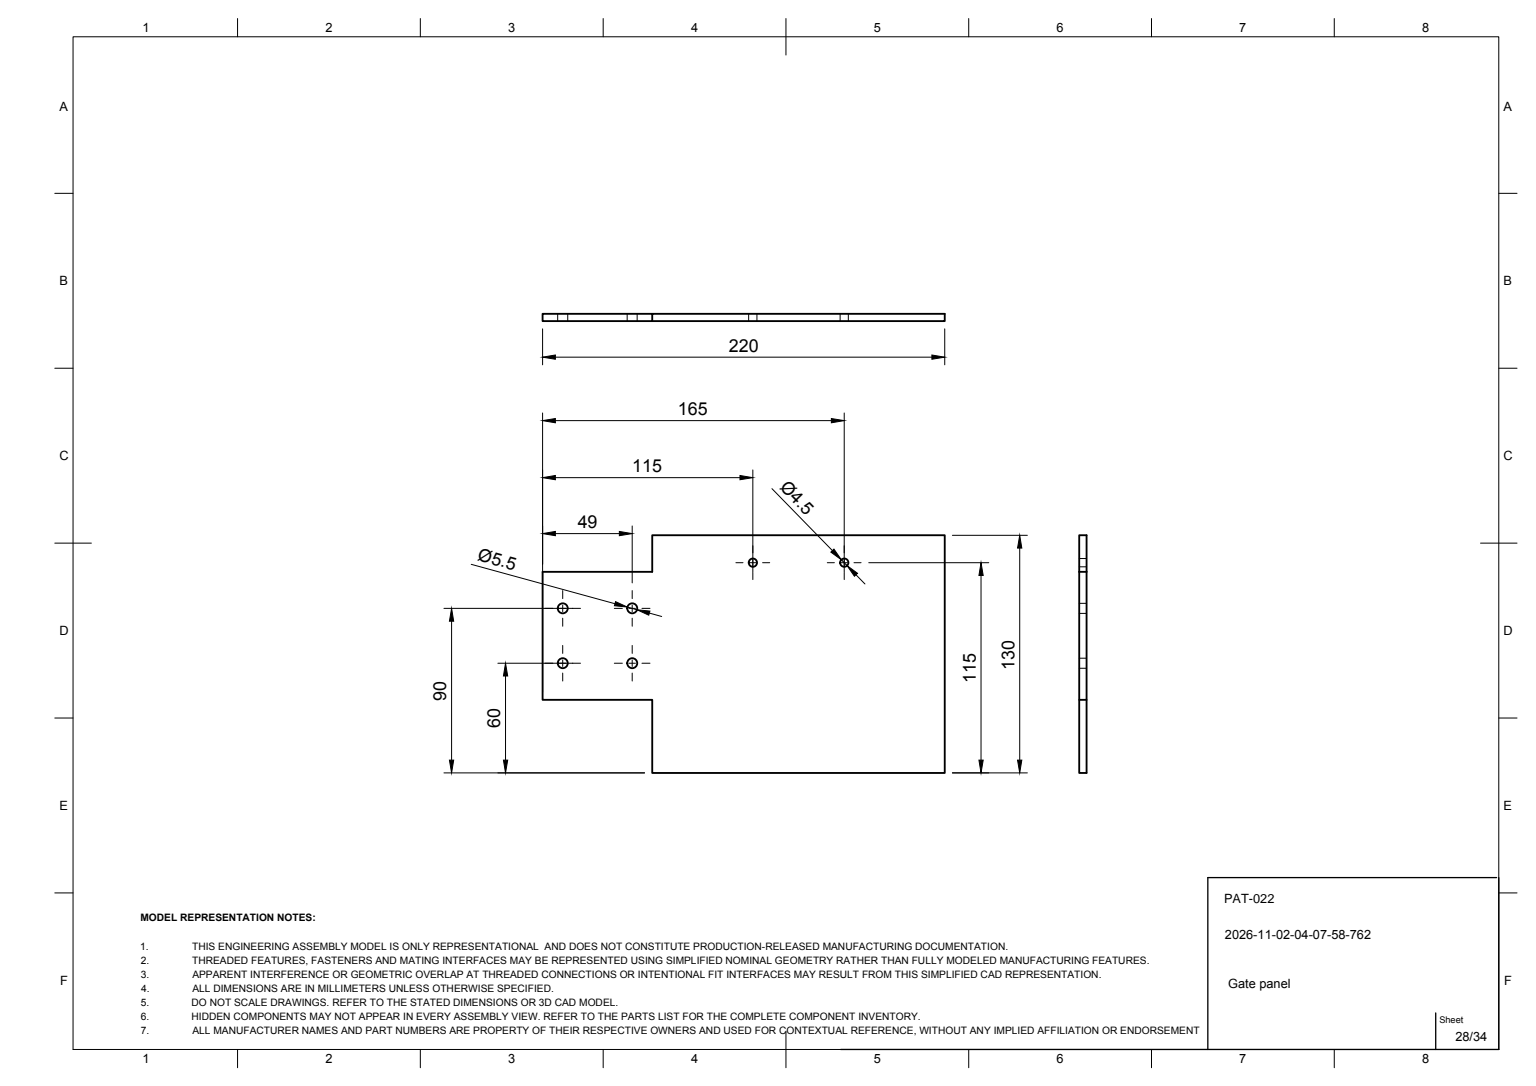
ISO-10303-21;
HEADER;
/* Generated by software containing ST-Developer
 * from STEP Tools, Inc. (www.steptools.com) 
 */

FILE_DESCRIPTION(
/* description */ ('Chute with adjustable gate'),
/* implementation_level */ '2;1');

FILE_NAME(
/* name */ 'Gate panel.step',
/* time_stamp */ '2026-10-27T10:52:28-07:00',
/* author */ (''),
/* organization */ (''),
/* preprocessor_version */ 'ST-DEVELOPER v20.2',
/* originating_system */ 'Autodesk Translation Framework v15.17.0.0',
/* authorisation */ '');

FILE_SCHEMA (('AUTOMOTIVE_DESIGN { 1 0 10303 214 3 1 1 }'));
ENDSEC;

DATA;
#10=MECHANICAL_DESIGN_GEOMETRIC_PRESENTATION_REPRESENTATION('',(#439),#13094);
#375=SHAPE_REPRESENTATION_RELATIONSHIP('SRR','None',#13277,#407);
#407=ADVANCED_BREP_SHAPE_REPRESENTATION('',(#469),#13086);
#439=STYLED_ITEM('',(#13488),#469);
#469=MANIFOLD_SOLID_BREP('Body1',#7624);
#570=FACE_BOUND('',#1746,.T.);
#571=FACE_BOUND('',#1747,.T.);
#572=FACE_BOUND('',#1748,.T.);
#573=FACE_BOUND('',#1749,.T.);
#574=FACE_BOUND('',#1750,.T.);
#575=FACE_BOUND('',#1751,.T.);
#576=FACE_BOUND('',#1758,.T.);
#577=FACE_BOUND('',#1759,.T.);
#578=FACE_BOUND('',#1760,.T.);
#579=FACE_BOUND('',#1761,.T.);
#580=FACE_BOUND('',#1762,.T.);
#581=FACE_BOUND('',#1763,.T.);
#836=PLANE('',#8470);
#837=PLANE('',#8471);
#838=PLANE('',#8472);
#839=PLANE('',#8473);
#840=PLANE('',#8474);
#841=PLANE('',#8475);
#842=PLANE('',#8476);
#843=PLANE('',#8477);
#844=PLANE('',#8478);
#845=PLANE('',#8479);
#1225=FACE_OUTER_BOUND('',#1736,.T.);
#1226=FACE_OUTER_BOUND('',#1737,.T.);
#1227=FACE_OUTER_BOUND('',#1738,.T.);
#1228=FACE_OUTER_BOUND('',#1739,.T.);
#1229=FACE_OUTER_BOUND('',#1740,.T.);
#1230=FACE_OUTER_BOUND('',#1741,.T.);
#1231=FACE_OUTER_BOUND('',#1742,.T.);
#1232=FACE_OUTER_BOUND('',#1743,.T.);
#1233=FACE_OUTER_BOUND('',#1744,.T.);
#1234=FACE_OUTER_BOUND('',#1745,.T.);
#1235=FACE_OUTER_BOUND('',#1752,.T.);
#1236=FACE_OUTER_BOUND('',#1753,.T.);
#1237=FACE_OUTER_BOUND('',#1754,.T.);
#1238=FACE_OUTER_BOUND('',#1755,.T.);
#1239=FACE_OUTER_BOUND('',#1756,.T.);
#1240=FACE_OUTER_BOUND('',#1757,.T.);
#1736=EDGE_LOOP('',(#6616,#6617,#6618,#6619));
#1737=EDGE_LOOP('',(#6620,#6621,#6622,#6623));
#1738=EDGE_LOOP('',(#6624,#6625,#6626,#6627));
#1739=EDGE_LOOP('',(#6628,#6629,#6630,#6631));
#1740=EDGE_LOOP('',(#6632,#6633,#6634,#6635));
#1741=EDGE_LOOP('',(#6636,#6637,#6638,#6639));
#1742=EDGE_LOOP('',(#6640,#6641,#6642,#6643));
#1743=EDGE_LOOP('',(#6644,#6645,#6646,#6647));
#1744=EDGE_LOOP('',(#6648,#6649,#6650,#6651));
#1745=EDGE_LOOP('',(#6652,#6653,#6654,#6655,#6656,#6657,#6658,#6659));
#1746=EDGE_LOOP('',(#6660));
#1747=EDGE_LOOP('',(#6661));
#1748=EDGE_LOOP('',(#6662));
#1749=EDGE_LOOP('',(#6663));
#1750=EDGE_LOOP('',(#6664));
#1751=EDGE_LOOP('',(#6665));
#1752=EDGE_LOOP('',(#6666,#6667,#6668,#6669));
#1753=EDGE_LOOP('',(#6670,#6671,#6672,#6673));
#1754=EDGE_LOOP('',(#6674,#6675,#6676,#6677));
#1755=EDGE_LOOP('',(#6678,#6679,#6680,#6681));
#1756=EDGE_LOOP('',(#6682,#6683,#6684,#6685));
#1757=EDGE_LOOP('',(#6686,#6687,#6688,#6689,#6690,#6691,#6692,#6693));
#1758=EDGE_LOOP('',(#6694));
#1759=EDGE_LOOP('',(#6695));
#1760=EDGE_LOOP('',(#6696));
#1761=EDGE_LOOP('',(#6697));
#1762=EDGE_LOOP('',(#6698));
#1763=EDGE_LOOP('',(#6699));
#2449=LINE('',#12432,#3226);
#2450=LINE('',#12438,#3227);
#2451=LINE('',#12444,#3228);
#2452=LINE('',#12450,#3229);
#2453=LINE('',#12456,#3230);
#2454=LINE('',#12462,#3231);
#2455=LINE('',#12467,#3232);
#2456=LINE('',#12469,#3233);
#2457=LINE('',#12471,#3234);
#2458=LINE('',#12472,#3235);
#2459=LINE('',#12476,#3236);
#2460=LINE('',#12478,#3237);
#2461=LINE('',#12480,#3238);
#2462=LINE('',#12481,#3239);
#2463=LINE('',#12483,#3240);
#2464=LINE('',#12484,#3241);
#2465=LINE('',#12487,#3242);
#2466=LINE('',#12489,#3243);
#2467=LINE('',#12491,#3244);
#2468=LINE('',#12493,#3245);
#2469=LINE('',#12494,#3246);
#2470=LINE('',#12497,#3247);
#2471=LINE('',#12498,#3248);
#2472=LINE('',#12501,#3249);
#2473=LINE('',#12503,#3250);
#2474=LINE('',#12504,#3251);
#2475=LINE('',#12506,#3252);
#2476=LINE('',#12509,#3253);
#2477=LINE('',#12510,#3254);
#2478=LINE('',#12512,#3255);
#3226=VECTOR('',#10223,0.225);
#3227=VECTOR('',#10230,0.225);
#3228=VECTOR('',#10237,0.275);
#3229=VECTOR('',#10244,0.275);
#3230=VECTOR('',#10251,0.275);
#3231=VECTOR('',#10258,0.275);
#3232=VECTOR('',#10263,1.);
#3233=VECTOR('',#10264,1.);
#3234=VECTOR('',#10265,1.);
#3235=VECTOR('',#10266,1.);
#3236=VECTOR('',#10269,1.);
#3237=VECTOR('',#10270,1.);
#3238=VECTOR('',#10271,1.);
#3239=VECTOR('',#10272,1.);
#3240=VECTOR('',#10275,1.);
#3241=VECTOR('',#10276,1.);
#3242=VECTOR('',#10279,1.);
#3243=VECTOR('',#10280,1.);
#3244=VECTOR('',#10281,1.);
#3245=VECTOR('',#10282,1.);
#3246=VECTOR('',#10283,1.);
#3247=VECTOR('',#10286,1.);
#3248=VECTOR('',#10287,1.);
#3249=VECTOR('',#10290,1.);
#3250=VECTOR('',#10291,1.);
#3251=VECTOR('',#10292,1.);
#3252=VECTOR('',#10295,1.);
#3253=VECTOR('',#10298,1.);
#3254=VECTOR('',#10299,1.);
#3255=VECTOR('',#10302,1.);
#3538=CIRCLE('',#8453,0.225);
#3539=CIRCLE('',#8454,0.225);
#3540=CIRCLE('',#8456,0.225);
#3541=CIRCLE('',#8457,0.225);
#3542=CIRCLE('',#8459,0.275);
#3543=CIRCLE('',#8460,0.275);
#3544=CIRCLE('',#8462,0.275);
#3545=CIRCLE('',#8463,0.275);
#3546=CIRCLE('',#8465,0.275);
#3547=CIRCLE('',#8466,0.275);
#3548=CIRCLE('',#8468,0.275);
#3549=CIRCLE('',#8469,0.275);
#4067=VERTEX_POINT('',#12429);
#4068=VERTEX_POINT('',#12431);
#4069=VERTEX_POINT('',#12435);
#4070=VERTEX_POINT('',#12437);
#4071=VERTEX_POINT('',#12441);
#4072=VERTEX_POINT('',#12443);
#4073=VERTEX_POINT('',#12447);
#4074=VERTEX_POINT('',#12449);
#4075=VERTEX_POINT('',#12453);
#4076=VERTEX_POINT('',#12455);
#4077=VERTEX_POINT('',#12459);
#4078=VERTEX_POINT('',#12461);
#4079=VERTEX_POINT('',#12465);
#4080=VERTEX_POINT('',#12466);
#4081=VERTEX_POINT('',#12468);
#4082=VERTEX_POINT('',#12470);
#4083=VERTEX_POINT('',#12474);
#4084=VERTEX_POINT('',#12475);
#4085=VERTEX_POINT('',#12477);
#4086=VERTEX_POINT('',#12479);
#4087=VERTEX_POINT('',#12486);
#4088=VERTEX_POINT('',#12488);
#4089=VERTEX_POINT('',#12490);
#4090=VERTEX_POINT('',#12492);
#4091=VERTEX_POINT('',#12496);
#4092=VERTEX_POINT('',#12500);
#4093=VERTEX_POINT('',#12502);
#4094=VERTEX_POINT('',#12508);
#4941=EDGE_CURVE('',#4067,#4067,#3538,.T.);
#4942=EDGE_CURVE('',#4067,#4068,#2449,.T.);
#4943=EDGE_CURVE('',#4068,#4068,#3539,.T.);
#4944=EDGE_CURVE('',#4069,#4069,#3540,.T.);
#4945=EDGE_CURVE('',#4069,#4070,#2450,.T.);
#4946=EDGE_CURVE('',#4070,#4070,#3541,.T.);
#4947=EDGE_CURVE('',#4071,#4071,#3542,.T.);
#4948=EDGE_CURVE('',#4071,#4072,#2451,.T.);
#4949=EDGE_CURVE('',#4072,#4072,#3543,.T.);
#4950=EDGE_CURVE('',#4073,#4073,#3544,.T.);
#4951=EDGE_CURVE('',#4073,#4074,#2452,.T.);
#4952=EDGE_CURVE('',#4074,#4074,#3545,.T.);
#4953=EDGE_CURVE('',#4075,#4075,#3546,.T.);
#4954=EDGE_CURVE('',#4075,#4076,#2453,.T.);
#4955=EDGE_CURVE('',#4076,#4076,#3547,.T.);
#4956=EDGE_CURVE('',#4077,#4077,#3548,.T.);
#4957=EDGE_CURVE('',#4077,#4078,#2454,.T.);
#4958=EDGE_CURVE('',#4078,#4078,#3549,.T.);
#4959=EDGE_CURVE('',#4079,#4080,#2455,.T.);
#4960=EDGE_CURVE('',#4081,#4079,#2456,.T.);
#4961=EDGE_CURVE('',#4082,#4081,#2457,.T.);
#4962=EDGE_CURVE('',#4082,#4080,#2458,.T.);
#4963=EDGE_CURVE('',#4083,#4084,#2459,.T.);
#4964=EDGE_CURVE('',#4083,#4085,#2460,.T.);
#4965=EDGE_CURVE('',#4085,#4086,#2461,.T.);
#4966=EDGE_CURVE('',#4084,#4086,#2462,.T.);
#4967=EDGE_CURVE('',#4085,#4082,#2463,.T.);
#4968=EDGE_CURVE('',#4086,#4081,#2464,.T.);
#4969=EDGE_CURVE('',#4087,#4083,#2465,.T.);
#4970=EDGE_CURVE('',#4088,#4087,#2466,.T.);
#4971=EDGE_CURVE('',#4089,#4088,#2467,.T.);
#4972=EDGE_CURVE('',#4090,#4089,#2468,.T.);
#4973=EDGE_CURVE('',#4080,#4090,#2469,.T.);
#4974=EDGE_CURVE('',#4091,#4084,#2470,.T.);
#4975=EDGE_CURVE('',#4087,#4091,#2471,.T.);
#4976=EDGE_CURVE('',#4089,#4092,#2472,.T.);
#4977=EDGE_CURVE('',#4093,#4092,#2473,.T.);
#4978=EDGE_CURVE('',#4090,#4093,#2474,.T.);
#4979=EDGE_CURVE('',#4079,#4093,#2475,.T.);
#4980=EDGE_CURVE('',#4094,#4091,#2476,.T.);
#4981=EDGE_CURVE('',#4088,#4094,#2477,.T.);
#4982=EDGE_CURVE('',#4092,#4094,#2478,.T.);
#6616=ORIENTED_EDGE('',*,*,#4941,.F.);
#6617=ORIENTED_EDGE('',*,*,#4942,.T.);
#6618=ORIENTED_EDGE('',*,*,#4943,.F.);
#6619=ORIENTED_EDGE('',*,*,#4942,.F.);
#6620=ORIENTED_EDGE('',*,*,#4944,.F.);
#6621=ORIENTED_EDGE('',*,*,#4945,.T.);
#6622=ORIENTED_EDGE('',*,*,#4946,.F.);
#6623=ORIENTED_EDGE('',*,*,#4945,.F.);
#6624=ORIENTED_EDGE('',*,*,#4947,.F.);
#6625=ORIENTED_EDGE('',*,*,#4948,.T.);
#6626=ORIENTED_EDGE('',*,*,#4949,.F.);
#6627=ORIENTED_EDGE('',*,*,#4948,.F.);
#6628=ORIENTED_EDGE('',*,*,#4950,.F.);
#6629=ORIENTED_EDGE('',*,*,#4951,.T.);
#6630=ORIENTED_EDGE('',*,*,#4952,.F.);
#6631=ORIENTED_EDGE('',*,*,#4951,.F.);
#6632=ORIENTED_EDGE('',*,*,#4953,.F.);
#6633=ORIENTED_EDGE('',*,*,#4954,.T.);
#6634=ORIENTED_EDGE('',*,*,#4955,.F.);
#6635=ORIENTED_EDGE('',*,*,#4954,.F.);
#6636=ORIENTED_EDGE('',*,*,#4956,.F.);
#6637=ORIENTED_EDGE('',*,*,#4957,.T.);
#6638=ORIENTED_EDGE('',*,*,#4958,.F.);
#6639=ORIENTED_EDGE('',*,*,#4957,.F.);
#6640=ORIENTED_EDGE('',*,*,#4959,.F.);
#6641=ORIENTED_EDGE('',*,*,#4960,.F.);
#6642=ORIENTED_EDGE('',*,*,#4961,.F.);
#6643=ORIENTED_EDGE('',*,*,#4962,.T.);
#6644=ORIENTED_EDGE('',*,*,#4963,.F.);
#6645=ORIENTED_EDGE('',*,*,#4964,.T.);
#6646=ORIENTED_EDGE('',*,*,#4965,.T.);
#6647=ORIENTED_EDGE('',*,*,#4966,.F.);
#6648=ORIENTED_EDGE('',*,*,#4967,.T.);
#6649=ORIENTED_EDGE('',*,*,#4961,.T.);
#6650=ORIENTED_EDGE('',*,*,#4968,.F.);
#6651=ORIENTED_EDGE('',*,*,#4965,.F.);
#6652=ORIENTED_EDGE('',*,*,#4969,.F.);
#6653=ORIENTED_EDGE('',*,*,#4970,.F.);
#6654=ORIENTED_EDGE('',*,*,#4971,.F.);
#6655=ORIENTED_EDGE('',*,*,#4972,.F.);
#6656=ORIENTED_EDGE('',*,*,#4973,.F.);
#6657=ORIENTED_EDGE('',*,*,#4962,.F.);
#6658=ORIENTED_EDGE('',*,*,#4967,.F.);
#6659=ORIENTED_EDGE('',*,*,#4964,.F.);
#6660=ORIENTED_EDGE('',*,*,#4941,.T.);
#6661=ORIENTED_EDGE('',*,*,#4944,.T.);
#6662=ORIENTED_EDGE('',*,*,#4947,.T.);
#6663=ORIENTED_EDGE('',*,*,#4950,.T.);
#6664=ORIENTED_EDGE('',*,*,#4953,.T.);
#6665=ORIENTED_EDGE('',*,*,#4956,.T.);
#6666=ORIENTED_EDGE('',*,*,#4963,.T.);
#6667=ORIENTED_EDGE('',*,*,#4974,.F.);
#6668=ORIENTED_EDGE('',*,*,#4975,.F.);
#6669=ORIENTED_EDGE('',*,*,#4969,.T.);
#6670=ORIENTED_EDGE('',*,*,#4972,.T.);
#6671=ORIENTED_EDGE('',*,*,#4976,.T.);
#6672=ORIENTED_EDGE('',*,*,#4977,.F.);
#6673=ORIENTED_EDGE('',*,*,#4978,.F.);
#6674=ORIENTED_EDGE('',*,*,#4959,.T.);
#6675=ORIENTED_EDGE('',*,*,#4973,.T.);
#6676=ORIENTED_EDGE('',*,*,#4978,.T.);
#6677=ORIENTED_EDGE('',*,*,#4979,.F.);
#6678=ORIENTED_EDGE('',*,*,#4970,.T.);
#6679=ORIENTED_EDGE('',*,*,#4975,.T.);
#6680=ORIENTED_EDGE('',*,*,#4980,.F.);
#6681=ORIENTED_EDGE('',*,*,#4981,.F.);
#6682=ORIENTED_EDGE('',*,*,#4971,.T.);
#6683=ORIENTED_EDGE('',*,*,#4981,.T.);
#6684=ORIENTED_EDGE('',*,*,#4982,.F.);
#6685=ORIENTED_EDGE('',*,*,#4976,.F.);
#6686=ORIENTED_EDGE('',*,*,#4979,.T.);
#6687=ORIENTED_EDGE('',*,*,#4977,.T.);
#6688=ORIENTED_EDGE('',*,*,#4982,.T.);
#6689=ORIENTED_EDGE('',*,*,#4980,.T.);
#6690=ORIENTED_EDGE('',*,*,#4974,.T.);
#6691=ORIENTED_EDGE('',*,*,#4966,.T.);
#6692=ORIENTED_EDGE('',*,*,#4968,.T.);
#6693=ORIENTED_EDGE('',*,*,#4960,.T.);
#6694=ORIENTED_EDGE('',*,*,#4943,.T.);
#6695=ORIENTED_EDGE('',*,*,#4946,.T.);
#6696=ORIENTED_EDGE('',*,*,#4949,.T.);
#6697=ORIENTED_EDGE('',*,*,#4952,.T.);
#6698=ORIENTED_EDGE('',*,*,#4955,.T.);
#6699=ORIENTED_EDGE('',*,*,#4958,.T.);
#7163=CYLINDRICAL_SURFACE('',#8452,0.225);
#7164=CYLINDRICAL_SURFACE('',#8455,0.225);
#7165=CYLINDRICAL_SURFACE('',#8458,0.275);
#7166=CYLINDRICAL_SURFACE('',#8461,0.275);
#7167=CYLINDRICAL_SURFACE('',#8464,0.275);
#7168=CYLINDRICAL_SURFACE('',#8467,0.275);
#7493=ADVANCED_FACE('',(#1225),#7163,.F.);
#7494=ADVANCED_FACE('',(#1226),#7164,.F.);
#7495=ADVANCED_FACE('',(#1227),#7165,.F.);
#7496=ADVANCED_FACE('',(#1228),#7166,.F.);
#7497=ADVANCED_FACE('',(#1229),#7167,.F.);
#7498=ADVANCED_FACE('',(#1230),#7168,.F.);
#7499=ADVANCED_FACE('',(#1231),#836,.T.);
#7500=ADVANCED_FACE('',(#1232),#837,.T.);
#7501=ADVANCED_FACE('',(#1233),#838,.T.);
#7502=ADVANCED_FACE('',(#1234,#570,#571,#572,#573,#574,#575),#839,.F.);
#7503=ADVANCED_FACE('',(#1235),#840,.T.);
#7504=ADVANCED_FACE('',(#1236),#841,.T.);
#7505=ADVANCED_FACE('',(#1237),#842,.T.);
#7506=ADVANCED_FACE('',(#1238),#843,.T.);
#7507=ADVANCED_FACE('',(#1239),#844,.T.);
#7508=ADVANCED_FACE('',(#1240,#576,#577,#578,#579,#580,#581),#845,.T.);
#7624=CLOSED_SHELL('',(#7493,#7494,#7495,#7496,#7497,#7498,#7499,#7500,
#7501,#7502,#7503,#7504,#7505,#7506,#7507,#7508));
#8451=AXIS2_PLACEMENT_3D('',#12427,#10217,#10218);
#8452=AXIS2_PLACEMENT_3D('',#12428,#10219,#10220);
#8453=AXIS2_PLACEMENT_3D('',#12430,#10221,#10222);
#8454=AXIS2_PLACEMENT_3D('',#12433,#10224,#10225);
#8455=AXIS2_PLACEMENT_3D('',#12434,#10226,#10227);
#8456=AXIS2_PLACEMENT_3D('',#12436,#10228,#10229);
#8457=AXIS2_PLACEMENT_3D('',#12439,#10231,#10232);
#8458=AXIS2_PLACEMENT_3D('',#12440,#10233,#10234);
#8459=AXIS2_PLACEMENT_3D('',#12442,#10235,#10236);
#8460=AXIS2_PLACEMENT_3D('',#12445,#10238,#10239);
#8461=AXIS2_PLACEMENT_3D('',#12446,#10240,#10241);
#8462=AXIS2_PLACEMENT_3D('',#12448,#10242,#10243);
#8463=AXIS2_PLACEMENT_3D('',#12451,#10245,#10246);
#8464=AXIS2_PLACEMENT_3D('',#12452,#10247,#10248);
#8465=AXIS2_PLACEMENT_3D('',#12454,#10249,#10250);
#8466=AXIS2_PLACEMENT_3D('',#12457,#10252,#10253);
#8467=AXIS2_PLACEMENT_3D('',#12458,#10254,#10255);
#8468=AXIS2_PLACEMENT_3D('',#12460,#10256,#10257);
#8469=AXIS2_PLACEMENT_3D('',#12463,#10259,#10260);
#8470=AXIS2_PLACEMENT_3D('',#12464,#10261,#10262);
#8471=AXIS2_PLACEMENT_3D('',#12473,#10267,#10268);
#8472=AXIS2_PLACEMENT_3D('',#12482,#10273,#10274);
#8473=AXIS2_PLACEMENT_3D('',#12485,#10277,#10278);
#8474=AXIS2_PLACEMENT_3D('',#12495,#10284,#10285);
#8475=AXIS2_PLACEMENT_3D('',#12499,#10288,#10289);
#8476=AXIS2_PLACEMENT_3D('',#12505,#10293,#10294);
#8477=AXIS2_PLACEMENT_3D('',#12507,#10296,#10297);
#8478=AXIS2_PLACEMENT_3D('',#12511,#10300,#10301);
#8479=AXIS2_PLACEMENT_3D('',#12513,#10303,#10304);
#10217=DIRECTION('axis',(0.,0.,1.));
#10218=DIRECTION('refdir',(1.,0.,0.));
#10219=DIRECTION('center_axis',(1.,0.,0.));
#10220=DIRECTION('ref_axis',(0.,0.,-1.));
#10221=DIRECTION('center_axis',(1.,0.,0.));
#10222=DIRECTION('ref_axis',(0.,0.,-1.));
#10223=DIRECTION('',(1.,0.,0.));
#10224=DIRECTION('center_axis',(-1.,0.,0.));
#10225=DIRECTION('ref_axis',(0.,0.,-1.));
#10226=DIRECTION('center_axis',(1.,0.,0.));
#10227=DIRECTION('ref_axis',(0.,0.,-1.));
#10228=DIRECTION('center_axis',(1.,0.,0.));
#10229=DIRECTION('ref_axis',(0.,0.,-1.));
#10230=DIRECTION('',(1.,0.,0.));
#10231=DIRECTION('center_axis',(-1.,0.,0.));
#10232=DIRECTION('ref_axis',(0.,0.,-1.));
#10233=DIRECTION('center_axis',(1.,0.,0.));
#10234=DIRECTION('ref_axis',(0.,0.,-1.));
#10235=DIRECTION('center_axis',(1.,0.,0.));
#10236=DIRECTION('ref_axis',(0.,0.,-1.));
#10237=DIRECTION('',(1.,0.,0.));
#10238=DIRECTION('center_axis',(-1.,0.,0.));
#10239=DIRECTION('ref_axis',(0.,0.,-1.));
#10240=DIRECTION('center_axis',(1.,0.,0.));
#10241=DIRECTION('ref_axis',(0.,0.,-1.));
#10242=DIRECTION('center_axis',(1.,0.,0.));
#10243=DIRECTION('ref_axis',(0.,0.,-1.));
#10244=DIRECTION('',(1.,0.,0.));
#10245=DIRECTION('center_axis',(-1.,0.,0.));
#10246=DIRECTION('ref_axis',(0.,0.,-1.));
#10247=DIRECTION('center_axis',(1.,0.,0.));
#10248=DIRECTION('ref_axis',(0.,0.,-1.));
#10249=DIRECTION('center_axis',(1.,0.,0.));
#10250=DIRECTION('ref_axis',(0.,0.,-1.));
#10251=DIRECTION('',(1.,0.,0.));
#10252=DIRECTION('center_axis',(-1.,0.,0.));
#10253=DIRECTION('ref_axis',(0.,0.,-1.));
#10254=DIRECTION('center_axis',(1.,0.,0.));
#10255=DIRECTION('ref_axis',(0.,0.,-1.));
#10256=DIRECTION('center_axis',(1.,0.,0.));
#10257=DIRECTION('ref_axis',(0.,0.,-1.));
#10258=DIRECTION('',(1.,0.,0.));
#10259=DIRECTION('center_axis',(-1.,0.,0.));
#10260=DIRECTION('ref_axis',(0.,0.,-1.));
#10261=DIRECTION('center_axis',(0.,0.,1.));
#10262=DIRECTION('ref_axis',(0.,-1.,0.));
#10263=DIRECTION('',(-1.,0.,0.));
#10264=DIRECTION('',(0.,-1.,0.));
#10265=DIRECTION('',(1.,0.,0.));
#10266=DIRECTION('',(0.,-1.,0.));
#10267=DIRECTION('center_axis',(0.,0.,-1.));
#10268=DIRECTION('ref_axis',(0.,1.,0.));
#10269=DIRECTION('',(1.,0.,0.));
#10270=DIRECTION('',(0.,1.,0.));
#10271=DIRECTION('',(1.,0.,0.));
#10272=DIRECTION('',(0.,1.,0.));
#10273=DIRECTION('center_axis',(0.,1.,0.));
#10274=DIRECTION('ref_axis',(0.,0.,1.));
#10275=DIRECTION('',(0.,0.,1.));
#10276=DIRECTION('',(0.,0.,1.));
#10277=DIRECTION('center_axis',(1.,0.,0.));
#10278=DIRECTION('ref_axis',(0.,0.,-1.));
#10279=DIRECTION('',(0.,0.,1.));
#10280=DIRECTION('',(0.,1.,0.));
#10281=DIRECTION('',(0.,0.,-1.));
#10282=DIRECTION('',(0.,-1.,0.));
#10283=DIRECTION('',(0.,0.,1.));
#10284=DIRECTION('center_axis',(0.,1.,0.));
#10285=DIRECTION('ref_axis',(0.,0.,1.));
#10286=DIRECTION('',(0.,0.,1.));
#10287=DIRECTION('',(1.,0.,0.));
#10288=DIRECTION('center_axis',(0.,0.,1.));
#10289=DIRECTION('ref_axis',(0.,-1.,0.));
#10290=DIRECTION('',(1.,0.,0.));
#10291=DIRECTION('',(0.,-1.,0.));
#10292=DIRECTION('',(1.,0.,0.));
#10293=DIRECTION('center_axis',(0.,1.,0.));
#10294=DIRECTION('ref_axis',(0.,0.,1.));
#10295=DIRECTION('',(0.,0.,1.));
#10296=DIRECTION('center_axis',(0.,0.,-1.));
#10297=DIRECTION('ref_axis',(0.,1.,0.));
#10298=DIRECTION('',(0.,1.,0.));
#10299=DIRECTION('',(1.,0.,0.));
#10300=DIRECTION('center_axis',(0.,-1.,0.));
#10301=DIRECTION('ref_axis',(0.,0.,-1.));
#10302=DIRECTION('',(0.,0.,-1.));
#10303=DIRECTION('center_axis',(1.,0.,0.));
#10304=DIRECTION('ref_axis',(0.,0.,-1.));
#12427=CARTESIAN_POINT('',(0.,0.,0.));
#12428=CARTESIAN_POINT('Origin',(-1.7,-2.5,15.));
#12429=CARTESIAN_POINT('',(-1.6,-2.5,15.225));
#12430=CARTESIAN_POINT('Origin',(-1.6,-2.5,15.));
#12431=CARTESIAN_POINT('',(-1.2,-2.5,15.225));
#12432=CARTESIAN_POINT('',(-1.7,-2.5,15.225));
#12433=CARTESIAN_POINT('Origin',(-1.2,-2.5,15.));
#12434=CARTESIAN_POINT('Origin',(-1.7,2.5,15.));
#12435=CARTESIAN_POINT('',(-1.6,2.5,15.225));
#12436=CARTESIAN_POINT('Origin',(-1.6,2.5,15.));
#12437=CARTESIAN_POINT('',(-1.2,2.5,15.225));
#12438=CARTESIAN_POINT('',(-1.7,2.5,15.225));
#12439=CARTESIAN_POINT('Origin',(-1.2,2.5,15.));
#12440=CARTESIAN_POINT('Origin',(-1.7,12.9,9.5));
#12441=CARTESIAN_POINT('',(-1.6,12.9,9.775));
#12442=CARTESIAN_POINT('Origin',(-1.6,12.9,9.5));
#12443=CARTESIAN_POINT('',(-1.2,12.9,9.775));
#12444=CARTESIAN_POINT('',(-1.7,12.9,9.775));
#12445=CARTESIAN_POINT('Origin',(-1.2,12.9,9.5));
#12446=CARTESIAN_POINT('Origin',(-1.7,9.1,12.5));
#12447=CARTESIAN_POINT('',(-1.6,9.1,12.775));
#12448=CARTESIAN_POINT('Origin',(-1.6,9.1,12.5));
#12449=CARTESIAN_POINT('',(-1.2,9.1,12.775));
#12450=CARTESIAN_POINT('',(-1.7,9.1,12.775));
#12451=CARTESIAN_POINT('Origin',(-1.2,9.1,12.5));
#12452=CARTESIAN_POINT('Origin',(-1.7,9.1,9.5));
#12453=CARTESIAN_POINT('',(-1.6,9.1,9.775));
#12454=CARTESIAN_POINT('Origin',(-1.6,9.1,9.5));
#12455=CARTESIAN_POINT('',(-1.2,9.1,9.775));
#12456=CARTESIAN_POINT('',(-1.7,9.1,9.775));
#12457=CARTESIAN_POINT('Origin',(-1.2,9.1,9.5));
#12458=CARTESIAN_POINT('Origin',(-1.7,12.9,12.5));
#12459=CARTESIAN_POINT('',(-1.6,12.9,12.775));
#12460=CARTESIAN_POINT('Origin',(-1.6,12.9,12.5));
#12461=CARTESIAN_POINT('',(-1.2,12.9,12.775));
#12462=CARTESIAN_POINT('',(-1.7,12.9,12.775));
#12463=CARTESIAN_POINT('Origin',(-1.2,12.9,12.5));
#12464=CARTESIAN_POINT('Origin',(-1.6,14.,14.5));
#12465=CARTESIAN_POINT('',(-1.2,8.,14.5));
#12466=CARTESIAN_POINT('',(-1.6,8.,14.5));
#12467=CARTESIAN_POINT('',(-1.6,8.,14.5));
#12468=CARTESIAN_POINT('',(-1.2,14.,14.5));
#12469=CARTESIAN_POINT('',(-1.2,14.,14.5));
#12470=CARTESIAN_POINT('',(-1.6,14.,14.5));
#12471=CARTESIAN_POINT('',(-1.6,14.,14.5));
#12472=CARTESIAN_POINT('',(-1.6,14.,14.5));
#12473=CARTESIAN_POINT('Origin',(-1.6,7.,7.5));
#12474=CARTESIAN_POINT('',(-1.6,8.,7.5));
#12475=CARTESIAN_POINT('',(-1.2,8.,7.5));
#12476=CARTESIAN_POINT('',(-1.6,8.,7.5));
#12477=CARTESIAN_POINT('',(-1.6,14.,7.5));
#12478=CARTESIAN_POINT('',(-1.6,7.,7.5));
#12479=CARTESIAN_POINT('',(-1.2,14.,7.5));
#12480=CARTESIAN_POINT('',(-1.6,14.,7.5));
#12481=CARTESIAN_POINT('',(-1.2,7.,7.5));
#12482=CARTESIAN_POINT('Origin',(-1.6,14.,7.5));
#12483=CARTESIAN_POINT('',(-1.6,14.,7.5));
#12484=CARTESIAN_POINT('',(-1.2,14.,7.5));
#12485=CARTESIAN_POINT('Origin',(-1.6,0.,10.));
#12486=CARTESIAN_POINT('',(-1.6,8.,3.5));
#12487=CARTESIAN_POINT('',(-1.6,8.,3.5));
#12488=CARTESIAN_POINT('',(-1.6,-8.,3.5));
#12489=CARTESIAN_POINT('',(-1.6,-8.,3.5));
#12490=CARTESIAN_POINT('',(-1.6,-8.,16.5));
#12491=CARTESIAN_POINT('',(-1.6,-8.,16.5));
#12492=CARTESIAN_POINT('',(-1.6,8.,16.5));
#12493=CARTESIAN_POINT('',(-1.6,8.,16.5));
#12494=CARTESIAN_POINT('',(-1.6,8.,3.5));
#12495=CARTESIAN_POINT('Origin',(-1.6,8.,3.5));
#12496=CARTESIAN_POINT('',(-1.2,8.,3.5));
#12497=CARTESIAN_POINT('',(-1.2,8.,3.5));
#12498=CARTESIAN_POINT('',(-1.6,8.,3.5));
#12499=CARTESIAN_POINT('Origin',(-1.6,8.,16.5));
#12500=CARTESIAN_POINT('',(-1.2,-8.,16.5));
#12501=CARTESIAN_POINT('',(-1.6,-8.,16.5));
#12502=CARTESIAN_POINT('',(-1.2,8.,16.5));
#12503=CARTESIAN_POINT('',(-1.2,8.,16.5));
#12504=CARTESIAN_POINT('',(-1.6,8.,16.5));
#12505=CARTESIAN_POINT('Origin',(-1.6,8.,3.5));
#12506=CARTESIAN_POINT('',(-1.2,8.,3.5));
#12507=CARTESIAN_POINT('Origin',(-1.6,-8.,3.5));
#12508=CARTESIAN_POINT('',(-1.2,-8.,3.5));
#12509=CARTESIAN_POINT('',(-1.2,-8.,3.5));
#12510=CARTESIAN_POINT('',(-1.6,-8.,3.5));
#12511=CARTESIAN_POINT('Origin',(-1.6,-8.,16.5));
#12512=CARTESIAN_POINT('',(-1.2,-8.,16.5));
#12513=CARTESIAN_POINT('Origin',(-1.2,0.,10.));
#13049=UNCERTAINTY_MEASURE_WITH_UNIT(LENGTH_MEASURE(0.001),#13095,
'DISTANCE_ACCURACY_VALUE',
'Maximum model space distance between geometric entities at asserted c
onnectivities');
#13057=UNCERTAINTY_MEASURE_WITH_UNIT(LENGTH_MEASURE(0.001),#13095,
'DISTANCE_ACCURACY_VALUE',
'Maximum model space distance between geometric entities at asserted c
onnectivities');
#13086=(
GEOMETRIC_REPRESENTATION_CONTEXT(3)
GLOBAL_UNCERTAINTY_ASSIGNED_CONTEXT((#13049))
GLOBAL_UNIT_ASSIGNED_CONTEXT((#13095,#13097,#13098))
REPRESENTATION_CONTEXT('','3D')
);
#13094=(
GEOMETRIC_REPRESENTATION_CONTEXT(3)
GLOBAL_UNCERTAINTY_ASSIGNED_CONTEXT((#13057))
GLOBAL_UNIT_ASSIGNED_CONTEXT((#13095,#13097,#13098))
REPRESENTATION_CONTEXT('','3D')
);
#13095=(
LENGTH_UNIT()
NAMED_UNIT(*)
SI_UNIT(.CENTI.,.METRE.)
);
#13097=(
NAMED_UNIT(*)
PLANE_ANGLE_UNIT()
SI_UNIT($,.RADIAN.)
);
#13098=(
NAMED_UNIT(*)
SI_UNIT($,.STERADIAN.)
SOLID_ANGLE_UNIT()
);
#13127=SHAPE_DEFINITION_REPRESENTATION(#13163,#13277);
#13163=PRODUCT_DEFINITION_SHAPE('',$,#13314);
#13277=SHAPE_REPRESENTATION('',(#8451),#13086);
#13285=PRODUCT_DEFINITION_CONTEXT('part definition',#13395,'design');
#13314=PRODUCT_DEFINITION('Gate panel','Gate panel',#13350,#13285);
#13350=PRODUCT_DEFINITION_FORMATION('',$,#13425);
#13395=APPLICATION_CONTEXT(
'Core Data for Automotive Mechanical Design Process');
#13396=PRODUCT_CONTEXT('part definition',#13395,'mechanical');
#13425=PRODUCT('Gate panel','Gate panel','Gate panel',(#13396));
#13482=COLOUR_RGB('Sky Blue',0.24,0.69,0.87);
#13483=FILL_AREA_STYLE_COLOUR('',#13482);
#13484=FILL_AREA_STYLE('',(#13483));
#13485=SURFACE_STYLE_FILL_AREA(#13484);
#13486=SURFACE_SIDE_STYLE('',(#13485));
#13487=SURFACE_STYLE_USAGE(.BOTH.,#13486);
#13488=PRESENTATION_STYLE_ASSIGNMENT((#13487));
ENDSEC;
END-ISO-10303-21;
